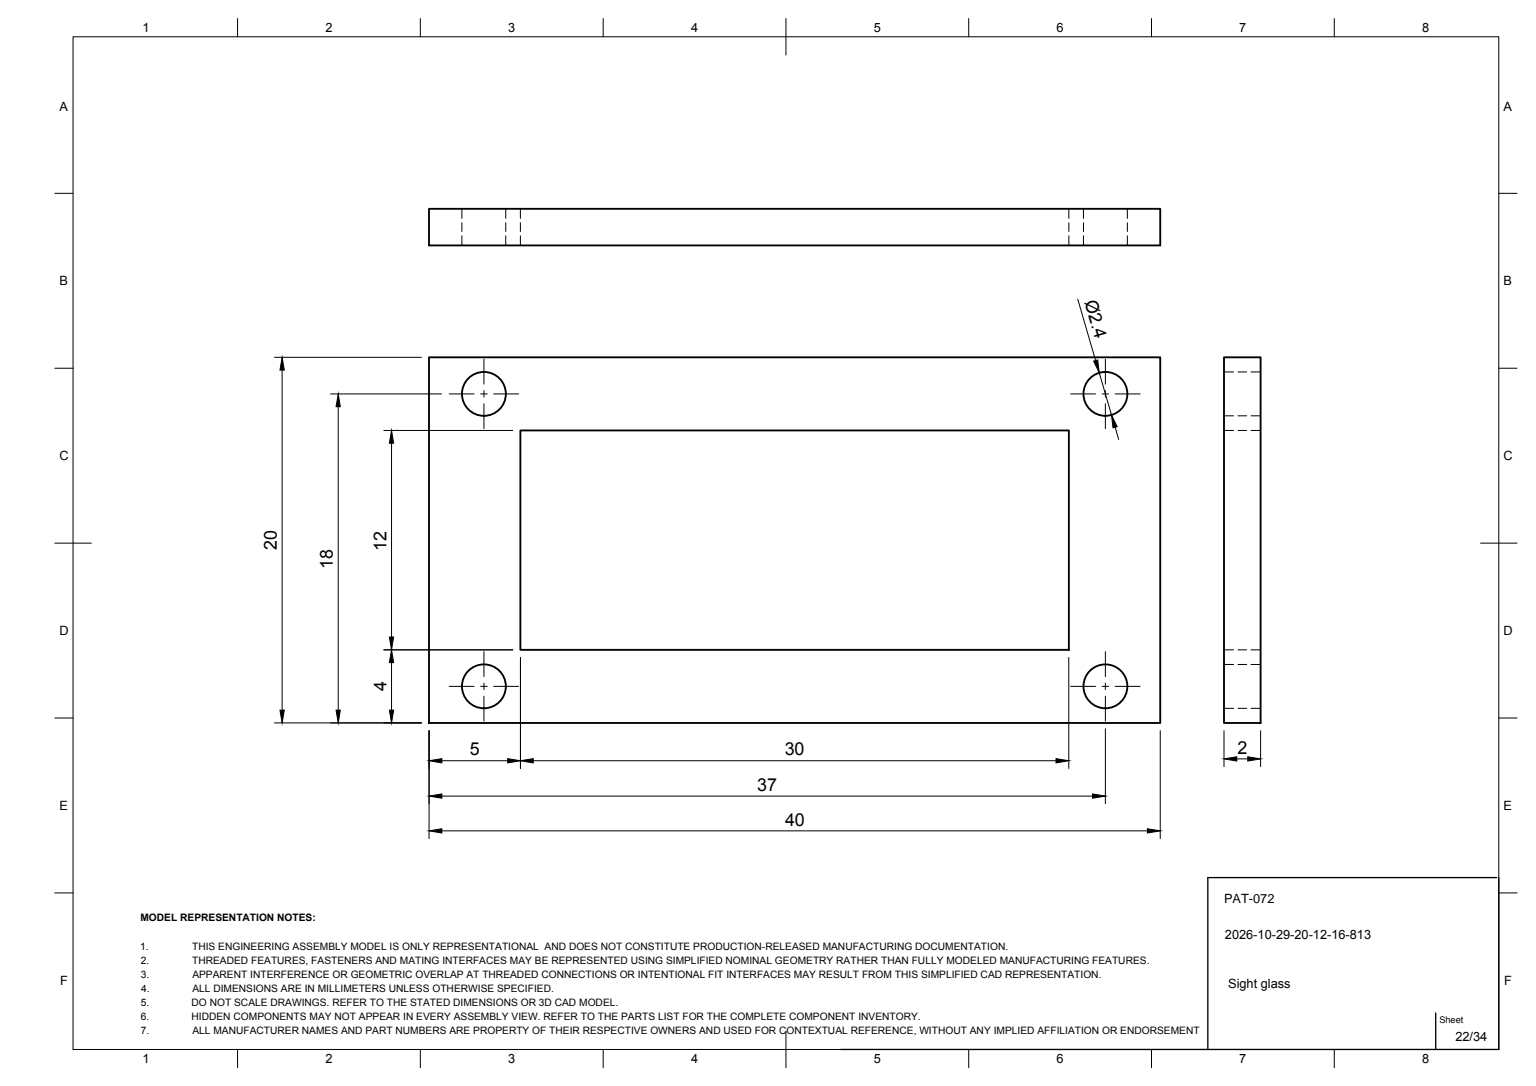
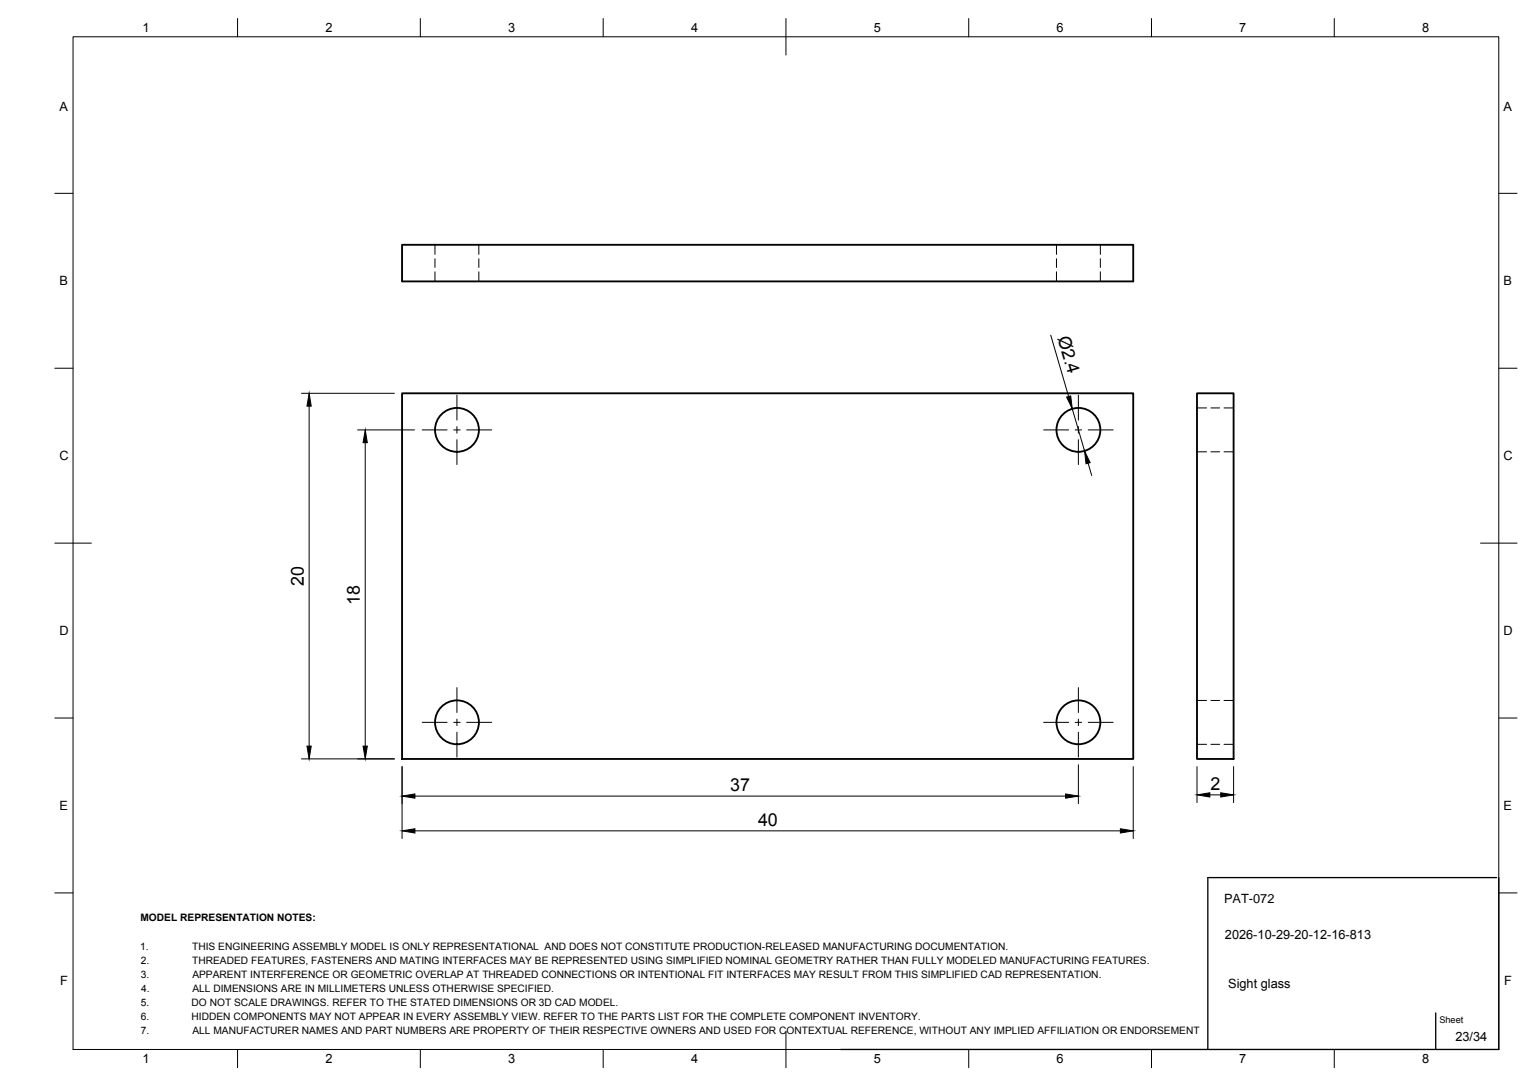
ISO-10303-21;
HEADER;
/* Generated by software containing ST-Developer
 * from STEP Tools, Inc. (www.steptools.com) 
 */

FILE_DESCRIPTION(
/* description */ ('PAT-072'),
/* implementation_level */ '2;1');

FILE_NAME(
/* name */ 'Sight glass.step',
/* time_stamp */ '2026-10-29T20:11:56-07:00',
/* author */ (''),
/* organization */ (''),
/* preprocessor_version */ 'ST-DEVELOPER v20.2',
/* originating_system */ 'Autodesk Translation Framework v15.17.0.0',
/* authorisation */ '');

FILE_SCHEMA (('AUTOMOTIVE_DESIGN { 1 0 10303 214 3 1 1 }'));
ENDSEC;

DATA;
#10=MECHANICAL_DESIGN_GEOMETRIC_PRESENTATION_REPRESENTATION('',(#352),#11432);
#280=SHAPE_REPRESENTATION_RELATIONSHIP('SRR','None',#11584,#316);
#316=ADVANCED_BREP_SHAPE_REPRESENTATION('',(#388),#11415);
#352=STYLED_ITEM('',(#11833),#388);
#388=MANIFOLD_SOLID_BREP('Body1',#6087);
#510=FACE_BOUND('',#1488,.T.);
#511=FACE_BOUND('',#1489,.T.);
#512=FACE_BOUND('',#1490,.T.);
#513=FACE_BOUND('',#1491,.T.);
#514=FACE_BOUND('',#1494,.T.);
#515=FACE_BOUND('',#1495,.T.);
#516=FACE_BOUND('',#1496,.T.);
#517=FACE_BOUND('',#1497,.T.);
#686=PLANE('',#6923);
#687=PLANE('',#6924);
#688=PLANE('',#6925);
#689=PLANE('',#6926);
#690=PLANE('',#6927);
#691=PLANE('',#6928);
#1003=FACE_OUTER_BOUND('',#1483,.T.);
#1004=FACE_OUTER_BOUND('',#1484,.T.);
#1005=FACE_OUTER_BOUND('',#1485,.T.);
#1006=FACE_OUTER_BOUND('',#1486,.T.);
#1007=FACE_OUTER_BOUND('',#1487,.T.);
#1008=FACE_OUTER_BOUND('',#1492,.T.);
#1009=FACE_OUTER_BOUND('',#1493,.T.);
#1010=FACE_OUTER_BOUND('',#1498,.T.);
#1011=FACE_OUTER_BOUND('',#1499,.T.);
#1012=FACE_OUTER_BOUND('',#1500,.T.);
#1483=EDGE_LOOP('',(#4886,#4887,#4888,#4889));
#1484=EDGE_LOOP('',(#4890,#4891,#4892,#4893));
#1485=EDGE_LOOP('',(#4894,#4895,#4896,#4897));
#1486=EDGE_LOOP('',(#4898,#4899,#4900,#4901));
#1487=EDGE_LOOP('',(#4902,#4903,#4904,#4905));
#1488=EDGE_LOOP('',(#4906));
#1489=EDGE_LOOP('',(#4907));
#1490=EDGE_LOOP('',(#4908));
#1491=EDGE_LOOP('',(#4909));
#1492=EDGE_LOOP('',(#4910,#4911,#4912,#4913));
#1493=EDGE_LOOP('',(#4914,#4915,#4916,#4917));
#1494=EDGE_LOOP('',(#4918));
#1495=EDGE_LOOP('',(#4919));
#1496=EDGE_LOOP('',(#4920));
#1497=EDGE_LOOP('',(#4921));
#1498=EDGE_LOOP('',(#4922,#4923,#4924,#4925));
#1499=EDGE_LOOP('',(#4926,#4927,#4928,#4929));
#1500=EDGE_LOOP('',(#4930,#4931,#4932,#4933));
#1908=LINE('',#10571,#2327);
#1909=LINE('',#10577,#2328);
#1910=LINE('',#10583,#2329);
#1911=LINE('',#10589,#2330);
#1912=LINE('',#10594,#2331);
#1913=LINE('',#10596,#2332);
#1914=LINE('',#10598,#2333);
#1915=LINE('',#10599,#2334);
#1916=LINE('',#10602,#2335);
#1917=LINE('',#10604,#2336);
#1918=LINE('',#10605,#2337);
#1919=LINE('',#10608,#2338);
#1920=LINE('',#10610,#2339);
#1921=LINE('',#10611,#2340);
#1922=LINE('',#10613,#2341);
#1923=LINE('',#10614,#2342);
#2327=VECTOR('',#8281,0.12);
#2328=VECTOR('',#8288,0.12);
#2329=VECTOR('',#8295,0.12);
#2330=VECTOR('',#8302,0.12);
#2331=VECTOR('',#8307,1.);
#2332=VECTOR('',#8308,1.);
#2333=VECTOR('',#8309,1.);
#2334=VECTOR('',#8310,1.);
#2335=VECTOR('',#8313,1.);
#2336=VECTOR('',#8314,1.);
#2337=VECTOR('',#8315,1.);
#2338=VECTOR('',#8318,1.);
#2339=VECTOR('',#8319,1.);
#2340=VECTOR('',#8320,1.);
#2341=VECTOR('',#8323,1.);
#2342=VECTOR('',#8324,1.);
#2719=CIRCLE('',#6912,0.12);
#2720=CIRCLE('',#6913,0.12);
#2721=CIRCLE('',#6915,0.12);
#2722=CIRCLE('',#6916,0.12);
#2723=CIRCLE('',#6918,0.12);
#2724=CIRCLE('',#6919,0.12);
#2725=CIRCLE('',#6921,0.12);
#2726=CIRCLE('',#6922,0.12);
#3102=VERTEX_POINT('',#10568);
#3103=VERTEX_POINT('',#10570);
#3104=VERTEX_POINT('',#10574);
#3105=VERTEX_POINT('',#10576);
#3106=VERTEX_POINT('',#10580);
#3107=VERTEX_POINT('',#10582);
#3108=VERTEX_POINT('',#10586);
#3109=VERTEX_POINT('',#10588);
#3110=VERTEX_POINT('',#10592);
#3111=VERTEX_POINT('',#10593);
#3112=VERTEX_POINT('',#10595);
#3113=VERTEX_POINT('',#10597);
#3114=VERTEX_POINT('',#10601);
#3115=VERTEX_POINT('',#10603);
#3116=VERTEX_POINT('',#10607);
#3117=VERTEX_POINT('',#10609);
#3732=EDGE_CURVE('',#3102,#3102,#2719,.T.);
#3733=EDGE_CURVE('',#3102,#3103,#1908,.T.);
#3734=EDGE_CURVE('',#3103,#3103,#2720,.T.);
#3735=EDGE_CURVE('',#3104,#3104,#2721,.T.);
#3736=EDGE_CURVE('',#3104,#3105,#1909,.T.);
#3737=EDGE_CURVE('',#3105,#3105,#2722,.T.);
#3738=EDGE_CURVE('',#3106,#3106,#2723,.T.);
#3739=EDGE_CURVE('',#3106,#3107,#1910,.T.);
#3740=EDGE_CURVE('',#3107,#3107,#2724,.T.);
#3741=EDGE_CURVE('',#3108,#3108,#2725,.T.);
#3742=EDGE_CURVE('',#3108,#3109,#1911,.T.);
#3743=EDGE_CURVE('',#3109,#3109,#2726,.T.);
#3744=EDGE_CURVE('',#3110,#3111,#1912,.T.);
#3745=EDGE_CURVE('',#3111,#3112,#1913,.T.);
#3746=EDGE_CURVE('',#3113,#3112,#1914,.T.);
#3747=EDGE_CURVE('',#3110,#3113,#1915,.T.);
#3748=EDGE_CURVE('',#3114,#3110,#1916,.T.);
#3749=EDGE_CURVE('',#3115,#3113,#1917,.T.);
#3750=EDGE_CURVE('',#3114,#3115,#1918,.T.);
#3751=EDGE_CURVE('',#3116,#3114,#1919,.T.);
#3752=EDGE_CURVE('',#3117,#3115,#1920,.T.);
#3753=EDGE_CURVE('',#3116,#3117,#1921,.T.);
#3754=EDGE_CURVE('',#3111,#3116,#1922,.T.);
#3755=EDGE_CURVE('',#3112,#3117,#1923,.T.);
#4886=ORIENTED_EDGE('',*,*,#3732,.F.);
#4887=ORIENTED_EDGE('',*,*,#3733,.T.);
#4888=ORIENTED_EDGE('',*,*,#3734,.F.);
#4889=ORIENTED_EDGE('',*,*,#3733,.F.);
#4890=ORIENTED_EDGE('',*,*,#3735,.F.);
#4891=ORIENTED_EDGE('',*,*,#3736,.T.);
#4892=ORIENTED_EDGE('',*,*,#3737,.F.);
#4893=ORIENTED_EDGE('',*,*,#3736,.F.);
#4894=ORIENTED_EDGE('',*,*,#3738,.F.);
#4895=ORIENTED_EDGE('',*,*,#3739,.T.);
#4896=ORIENTED_EDGE('',*,*,#3740,.F.);
#4897=ORIENTED_EDGE('',*,*,#3739,.F.);
#4898=ORIENTED_EDGE('',*,*,#3741,.F.);
#4899=ORIENTED_EDGE('',*,*,#3742,.T.);
#4900=ORIENTED_EDGE('',*,*,#3743,.F.);
#4901=ORIENTED_EDGE('',*,*,#3742,.F.);
#4902=ORIENTED_EDGE('',*,*,#3744,.T.);
#4903=ORIENTED_EDGE('',*,*,#3745,.T.);
#4904=ORIENTED_EDGE('',*,*,#3746,.F.);
#4905=ORIENTED_EDGE('',*,*,#3747,.F.);
#4906=ORIENTED_EDGE('',*,*,#3734,.T.);
#4907=ORIENTED_EDGE('',*,*,#3737,.T.);
#4908=ORIENTED_EDGE('',*,*,#3740,.T.);
#4909=ORIENTED_EDGE('',*,*,#3743,.T.);
#4910=ORIENTED_EDGE('',*,*,#3748,.T.);
#4911=ORIENTED_EDGE('',*,*,#3747,.T.);
#4912=ORIENTED_EDGE('',*,*,#3749,.F.);
#4913=ORIENTED_EDGE('',*,*,#3750,.F.);
#4914=ORIENTED_EDGE('',*,*,#3751,.T.);
#4915=ORIENTED_EDGE('',*,*,#3750,.T.);
#4916=ORIENTED_EDGE('',*,*,#3752,.F.);
#4917=ORIENTED_EDGE('',*,*,#3753,.F.);
#4918=ORIENTED_EDGE('',*,*,#3732,.T.);
#4919=ORIENTED_EDGE('',*,*,#3735,.T.);
#4920=ORIENTED_EDGE('',*,*,#3738,.T.);
#4921=ORIENTED_EDGE('',*,*,#3741,.T.);
#4922=ORIENTED_EDGE('',*,*,#3754,.T.);
#4923=ORIENTED_EDGE('',*,*,#3753,.T.);
#4924=ORIENTED_EDGE('',*,*,#3755,.F.);
#4925=ORIENTED_EDGE('',*,*,#3745,.F.);
#4926=ORIENTED_EDGE('',*,*,#3755,.T.);
#4927=ORIENTED_EDGE('',*,*,#3752,.T.);
#4928=ORIENTED_EDGE('',*,*,#3749,.T.);
#4929=ORIENTED_EDGE('',*,*,#3746,.T.);
#4930=ORIENTED_EDGE('',*,*,#3754,.F.);
#4931=ORIENTED_EDGE('',*,*,#3744,.F.);
#4932=ORIENTED_EDGE('',*,*,#3748,.F.);
#4933=ORIENTED_EDGE('',*,*,#3751,.F.);
#5649=CYLINDRICAL_SURFACE('',#6911,0.12);
#5650=CYLINDRICAL_SURFACE('',#6914,0.12);
#5651=CYLINDRICAL_SURFACE('',#6917,0.12);
#5652=CYLINDRICAL_SURFACE('',#6920,0.12);
#5902=ADVANCED_FACE('',(#1003),#5649,.F.);
#5903=ADVANCED_FACE('',(#1004),#5650,.F.);
#5904=ADVANCED_FACE('',(#1005),#5651,.F.);
#5905=ADVANCED_FACE('',(#1006),#5652,.F.);
#5906=ADVANCED_FACE('',(#1007,#510,#511,#512,#513),#686,.T.);
#5907=ADVANCED_FACE('',(#1008),#687,.T.);
#5908=ADVANCED_FACE('',(#1009,#514,#515,#516,#517),#688,.T.);
#5909=ADVANCED_FACE('',(#1010),#689,.T.);
#5910=ADVANCED_FACE('',(#1011),#690,.T.);
#5911=ADVANCED_FACE('',(#1012),#691,.F.);
#6087=CLOSED_SHELL('',(#5902,#5903,#5904,#5905,#5906,#5907,#5908,#5909,
#5910,#5911));
#6910=AXIS2_PLACEMENT_3D('',#10566,#8275,#8276);
#6911=AXIS2_PLACEMENT_3D('',#10567,#8277,#8278);
#6912=AXIS2_PLACEMENT_3D('',#10569,#8279,#8280);
#6913=AXIS2_PLACEMENT_3D('',#10572,#8282,#8283);
#6914=AXIS2_PLACEMENT_3D('',#10573,#8284,#8285);
#6915=AXIS2_PLACEMENT_3D('',#10575,#8286,#8287);
#6916=AXIS2_PLACEMENT_3D('',#10578,#8289,#8290);
#6917=AXIS2_PLACEMENT_3D('',#10579,#8291,#8292);
#6918=AXIS2_PLACEMENT_3D('',#10581,#8293,#8294);
#6919=AXIS2_PLACEMENT_3D('',#10584,#8296,#8297);
#6920=AXIS2_PLACEMENT_3D('',#10585,#8298,#8299);
#6921=AXIS2_PLACEMENT_3D('',#10587,#8300,#8301);
#6922=AXIS2_PLACEMENT_3D('',#10590,#8303,#8304);
#6923=AXIS2_PLACEMENT_3D('',#10591,#8305,#8306);
#6924=AXIS2_PLACEMENT_3D('',#10600,#8311,#8312);
#6925=AXIS2_PLACEMENT_3D('',#10606,#8316,#8317);
#6926=AXIS2_PLACEMENT_3D('',#10612,#8321,#8322);
#6927=AXIS2_PLACEMENT_3D('',#10615,#8325,#8326);
#6928=AXIS2_PLACEMENT_3D('',#10616,#8327,#8328);
#8275=DIRECTION('axis',(0.,0.,1.));
#8276=DIRECTION('refdir',(1.,0.,0.));
#8277=DIRECTION('center_axis',(0.,1.,0.));
#8278=DIRECTION('ref_axis',(1.,0.,0.));
#8279=DIRECTION('center_axis',(0.,1.,0.));
#8280=DIRECTION('ref_axis',(1.,0.,0.));
#8281=DIRECTION('',(0.,1.,0.));
#8282=DIRECTION('center_axis',(0.,-1.,0.));
#8283=DIRECTION('ref_axis',(1.,0.,0.));
#8284=DIRECTION('center_axis',(0.,1.,0.));
#8285=DIRECTION('ref_axis',(1.,0.,0.));
#8286=DIRECTION('center_axis',(0.,1.,0.));
#8287=DIRECTION('ref_axis',(1.,0.,0.));
#8288=DIRECTION('',(0.,1.,0.));
#8289=DIRECTION('center_axis',(0.,-1.,0.));
#8290=DIRECTION('ref_axis',(1.,0.,0.));
#8291=DIRECTION('center_axis',(0.,1.,0.));
#8292=DIRECTION('ref_axis',(1.,0.,0.));
#8293=DIRECTION('center_axis',(0.,1.,0.));
#8294=DIRECTION('ref_axis',(1.,0.,0.));
#8295=DIRECTION('',(0.,1.,0.));
#8296=DIRECTION('center_axis',(0.,-1.,0.));
#8297=DIRECTION('ref_axis',(1.,0.,0.));
#8298=DIRECTION('center_axis',(0.,1.,0.));
#8299=DIRECTION('ref_axis',(1.,0.,0.));
#8300=DIRECTION('center_axis',(0.,1.,0.));
#8301=DIRECTION('ref_axis',(1.,0.,0.));
#8302=DIRECTION('',(0.,1.,0.));
#8303=DIRECTION('center_axis',(0.,-1.,0.));
#8304=DIRECTION('ref_axis',(1.,0.,0.));
#8305=DIRECTION('center_axis',(0.,1.,0.));
#8306=DIRECTION('ref_axis',(-1.,0.,0.));
#8307=DIRECTION('',(-1.,0.,0.));
#8308=DIRECTION('',(0.,0.,1.));
#8309=DIRECTION('',(-1.,0.,0.));
#8310=DIRECTION('',(0.,0.,1.));
#8311=DIRECTION('center_axis',(1.,0.,0.));
#8312=DIRECTION('ref_axis',(0.,1.,0.));
#8313=DIRECTION('',(0.,1.,0.));
#8314=DIRECTION('',(0.,1.,0.));
#8315=DIRECTION('',(0.,0.,1.));
#8316=DIRECTION('center_axis',(0.,-1.,0.));
#8317=DIRECTION('ref_axis',(1.,0.,0.));
#8318=DIRECTION('',(1.,0.,0.));
#8319=DIRECTION('',(1.,0.,0.));
#8320=DIRECTION('',(0.,0.,1.));
#8321=DIRECTION('center_axis',(-1.,0.,0.));
#8322=DIRECTION('ref_axis',(0.,-1.,0.));
#8323=DIRECTION('',(0.,-1.,0.));
#8324=DIRECTION('',(0.,-1.,0.));
#8325=DIRECTION('center_axis',(0.,0.,1.));
#8326=DIRECTION('ref_axis',(1.,0.,0.));
#8327=DIRECTION('center_axis',(0.,0.,1.));
#8328=DIRECTION('ref_axis',(1.,0.,0.));
#10566=CARTESIAN_POINT('',(0.,0.,0.));
#10567=CARTESIAN_POINT('Origin',(0.8,-3.2,9.8));
#10568=CARTESIAN_POINT('',(0.68,-2.9,9.8));
#10569=CARTESIAN_POINT('Origin',(0.8,-2.9,9.8));
#10570=CARTESIAN_POINT('',(0.68,-2.7,9.8));
#10571=CARTESIAN_POINT('',(0.68,-3.2,9.8));
#10572=CARTESIAN_POINT('Origin',(0.8,-2.7,9.8));
#10573=CARTESIAN_POINT('Origin',(-0.8,-3.2,13.2));
#10574=CARTESIAN_POINT('',(-0.92,-2.9,13.2));
#10575=CARTESIAN_POINT('Origin',(-0.8,-2.9,13.2));
#10576=CARTESIAN_POINT('',(-0.92,-2.7,13.2));
#10577=CARTESIAN_POINT('',(-0.92,-3.2,13.2));
#10578=CARTESIAN_POINT('Origin',(-0.8,-2.7,13.2));
#10579=CARTESIAN_POINT('Origin',(-0.8,-3.2,9.8));
#10580=CARTESIAN_POINT('',(-0.92,-2.9,9.8));
#10581=CARTESIAN_POINT('Origin',(-0.8,-2.9,9.8));
#10582=CARTESIAN_POINT('',(-0.92,-2.7,9.8));
#10583=CARTESIAN_POINT('',(-0.92,-3.2,9.8));
#10584=CARTESIAN_POINT('Origin',(-0.8,-2.7,9.8));
#10585=CARTESIAN_POINT('Origin',(0.8,-3.2,13.2));
#10586=CARTESIAN_POINT('',(0.68,-2.9,13.2));
#10587=CARTESIAN_POINT('Origin',(0.8,-2.9,13.2));
#10588=CARTESIAN_POINT('',(0.68,-2.7,13.2));
#10589=CARTESIAN_POINT('',(0.68,-3.2,13.2));
#10590=CARTESIAN_POINT('Origin',(0.8,-2.7,13.2));
#10591=CARTESIAN_POINT('Origin',(1.,-2.7,9.5));
#10592=CARTESIAN_POINT('',(1.,-2.7,9.5));
#10593=CARTESIAN_POINT('',(-1.,-2.7,9.5));
#10594=CARTESIAN_POINT('',(1.,-2.7,9.5));
#10595=CARTESIAN_POINT('',(-1.,-2.7,13.5));
#10596=CARTESIAN_POINT('',(-1.,-2.7,9.5));
#10597=CARTESIAN_POINT('',(1.,-2.7,13.5));
#10598=CARTESIAN_POINT('',(1.,-2.7,13.5));
#10599=CARTESIAN_POINT('',(1.,-2.7,9.5));
#10600=CARTESIAN_POINT('Origin',(1.,-2.9,9.5));
#10601=CARTESIAN_POINT('',(1.,-2.9,9.5));
#10602=CARTESIAN_POINT('',(1.,-2.9,9.5));
#10603=CARTESIAN_POINT('',(1.,-2.9,13.5));
#10604=CARTESIAN_POINT('',(1.,-2.9,13.5));
#10605=CARTESIAN_POINT('',(1.,-2.9,9.5));
#10606=CARTESIAN_POINT('Origin',(-1.,-2.9,9.5));
#10607=CARTESIAN_POINT('',(-1.,-2.9,9.5));
#10608=CARTESIAN_POINT('',(-1.,-2.9,9.5));
#10609=CARTESIAN_POINT('',(-1.,-2.9,13.5));
#10610=CARTESIAN_POINT('',(-1.,-2.9,13.5));
#10611=CARTESIAN_POINT('',(-1.,-2.9,9.5));
#10612=CARTESIAN_POINT('Origin',(-1.,-2.7,9.5));
#10613=CARTESIAN_POINT('',(-1.,-2.7,9.5));
#10614=CARTESIAN_POINT('',(-1.,-2.7,13.5));
#10615=CARTESIAN_POINT('Origin',(0.,-2.8,13.5));
#10616=CARTESIAN_POINT('Origin',(0.,-2.8,9.5));
#11376=UNCERTAINTY_MEASURE_WITH_UNIT(LENGTH_MEASURE(0.001),#11433,
'DISTANCE_ACCURACY_VALUE',
'Maximum model space distance between geometric entities at asserted c
onnectivities');
#11393=UNCERTAINTY_MEASURE_WITH_UNIT(LENGTH_MEASURE(0.001),#11433,
'DISTANCE_ACCURACY_VALUE',
'Maximum model space distance between geometric entities at asserted c
onnectivities');
#11415=(
GEOMETRIC_REPRESENTATION_CONTEXT(3)
GLOBAL_UNCERTAINTY_ASSIGNED_CONTEXT((#11376))
GLOBAL_UNIT_ASSIGNED_CONTEXT((#11433,#11435,#11436))
REPRESENTATION_CONTEXT('','3D')
);
#11432=(
GEOMETRIC_REPRESENTATION_CONTEXT(3)
GLOBAL_UNCERTAINTY_ASSIGNED_CONTEXT((#11393))
GLOBAL_UNIT_ASSIGNED_CONTEXT((#11433,#11435,#11436))
REPRESENTATION_CONTEXT('','3D')
);
#11433=(
LENGTH_UNIT()
NAMED_UNIT(*)
SI_UNIT(.CENTI.,.METRE.)
);
#11435=(
NAMED_UNIT(*)
PLANE_ANGLE_UNIT()
SI_UNIT($,.RADIAN.)
);
#11436=(
NAMED_UNIT(*)
SI_UNIT($,.STERADIAN.)
SOLID_ANGLE_UNIT()
);
#11458=SHAPE_DEFINITION_REPRESENTATION(#11496,#11584);
#11496=PRODUCT_DEFINITION_SHAPE('',$,#11623);
#11584=SHAPE_REPRESENTATION('',(#6910),#11415);
#11601=PRODUCT_DEFINITION_CONTEXT('part definition',#11717,'design');
#11623=PRODUCT_DEFINITION('Sight glass','Sight glass',#11661,
#11601);
#11661=PRODUCT_DEFINITION_FORMATION('',$,#11740);
#11717=APPLICATION_CONTEXT(
'Core Data for Automotive Mechanical Design Process');
#11718=PRODUCT_CONTEXT('part definition',#11717,'mechanical');
#11740=PRODUCT('Sight glass','Sight glass','Sight glass',(#11718));
#11827=COLOUR_RGB('Off White',0.89,0.88,0.83);
#11828=FILL_AREA_STYLE_COLOUR('',#11827);
#11829=FILL_AREA_STYLE('',(#11828));
#11830=SURFACE_STYLE_FILL_AREA(#11829);
#11831=SURFACE_SIDE_STYLE('',(#11830));
#11832=SURFACE_STYLE_USAGE(.BOTH.,#11831);
#11833=PRESENTATION_STYLE_ASSIGNMENT((#11832));
ENDSEC;
END-ISO-10303-21;
